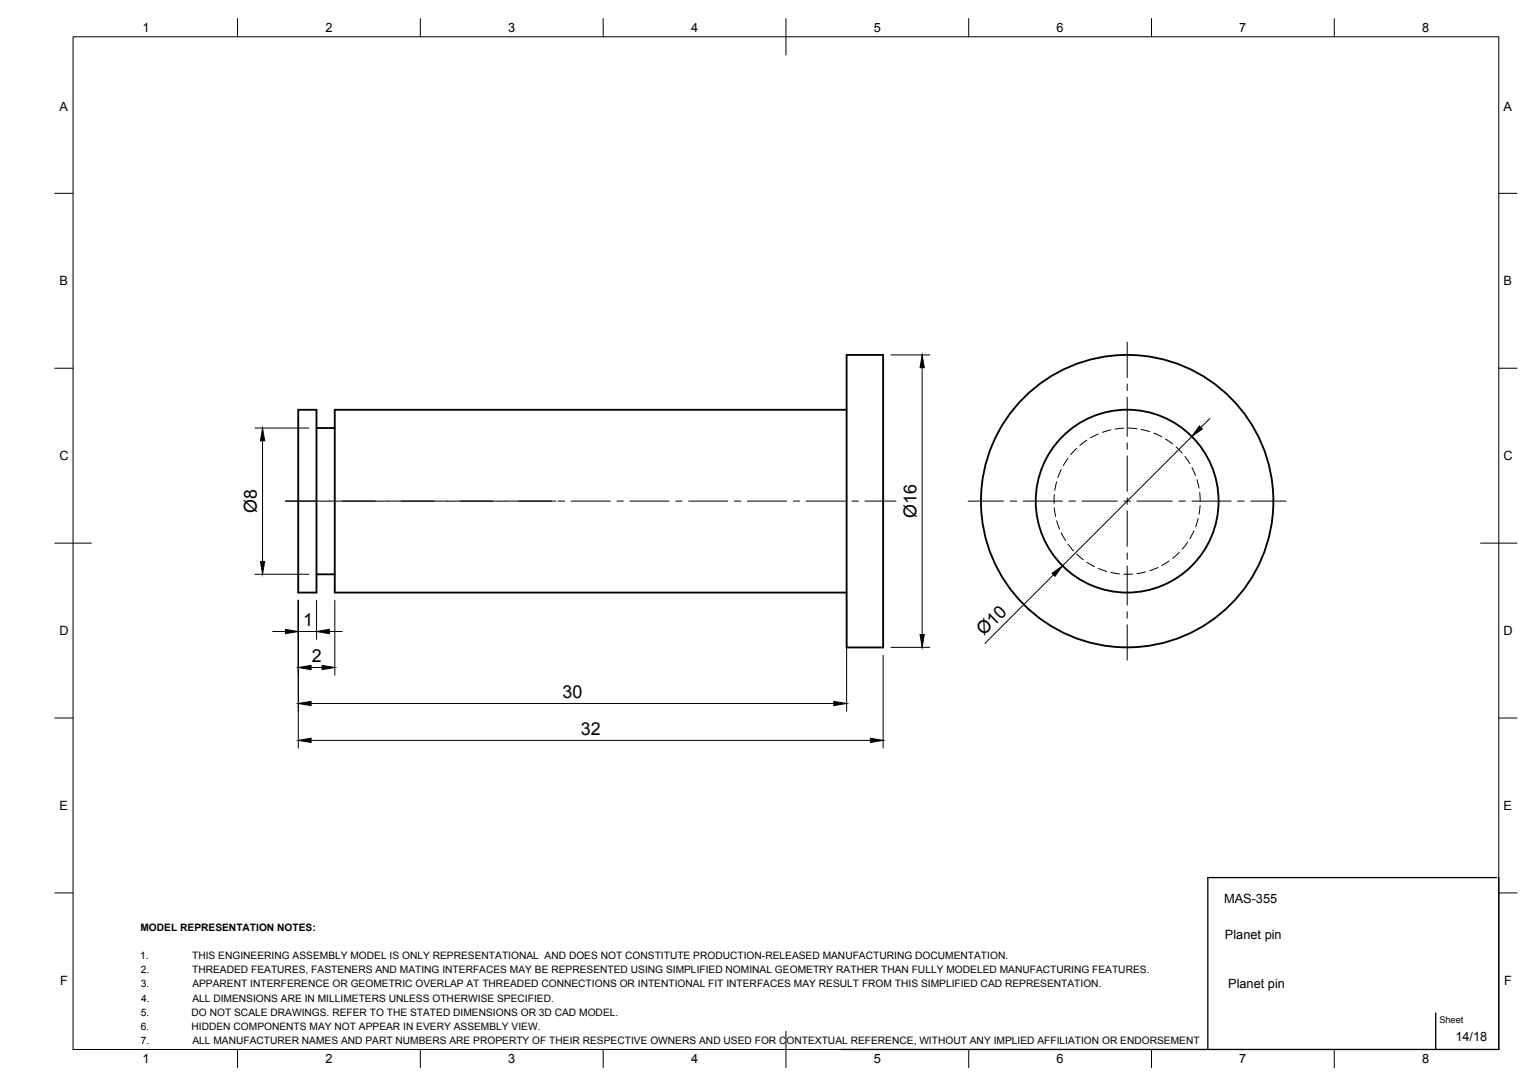
ISO-10303-21;
HEADER;
/* Generated by software containing ST-Developer
 * from STEP Tools, Inc. (www.steptools.com) 
 */

FILE_DESCRIPTION(
/* description */ ('Independent two-stage fixed-ring planetary gearbox,24/24/72 teeth,mod
ule2,20deg involutes,three planets per stage,4:1 x4:1=16:1. Native cut
-space/fillet/pattern tooth profiles derived from reusable gear blanks
; shared sun/planet/ring/carrier parts across both stages. Captured br
onze-journal input/carriers, headed retained planet pins, keyed inters
tage drive and modular keyed output interface. Native ideal gear links
; no torque, precision grade, production backlash/fits, lubrication, s
peed or life rating.'),
/* implementation_level */ '2;1');

FILE_NAME(
/* name */ 'Planet pin.step',
/* time_stamp */ '2026-11-08T19:10:00-08:00',
/* author */ (''),
/* organization */ (''),
/* preprocessor_version */ 'ST-DEVELOPER v20.2',
/* originating_system */ 'Autodesk Translation Framework v15.17.0.0',
/* authorisation */ '');

FILE_SCHEMA (('AUTOMOTIVE_DESIGN { 1 0 10303 214 3 1 1 }'));
ENDSEC;

DATA;
#10=MECHANICAL_DESIGN_GEOMETRIC_PRESENTATION_REPRESENTATION('',(#1174),#259224);
#1134=SHAPE_REPRESENTATION_RELATIONSHIP('SRR','None',#259381,#1154);
#1154=ADVANCED_BREP_SHAPE_REPRESENTATION('',(#1194),#259215);
#1174=STYLED_ITEM('',(#259488),#1194);
#1194=MANIFOLD_SOLID_BREP('Body1',#25161);
#1307=FACE_BOUND('',#4399,.T.);
#1308=FACE_BOUND('',#4401,.T.);
#1309=FACE_BOUND('',#4404,.T.);
#1663=PLANE('',#27096);
#1664=PLANE('',#27098);
#1665=PLANE('',#27102);
#1666=PLANE('',#27107);
#1667=PLANE('',#27109);
#2947=FACE_OUTER_BOUND('',#4397,.T.);
#2948=FACE_OUTER_BOUND('',#4398,.T.);
#2949=FACE_OUTER_BOUND('',#4400,.T.);
#2950=FACE_OUTER_BOUND('',#4402,.T.);
#2951=FACE_OUTER_BOUND('',#4403,.T.);
#2952=FACE_OUTER_BOUND('',#4405,.T.);
#2953=FACE_OUTER_BOUND('',#4406,.T.);
#2954=FACE_OUTER_BOUND('',#4407,.T.);
#2955=FACE_OUTER_BOUND('',#4408,.T.);
#4397=EDGE_LOOP('',(#22634,#22635,#22636,#22637));
#4398=EDGE_LOOP('',(#22638));
#4399=EDGE_LOOP('',(#22639));
#4400=EDGE_LOOP('',(#22640));
#4401=EDGE_LOOP('',(#22641));
#4402=EDGE_LOOP('',(#22642,#22643,#22644,#22645));
#4403=EDGE_LOOP('',(#22646));
#4404=EDGE_LOOP('',(#22647));
#4405=EDGE_LOOP('',(#22648,#22649,#22650,#22651));
#4406=EDGE_LOOP('',(#22652));
#4407=EDGE_LOOP('',(#22653,#22654,#22655,#22656));
#4408=EDGE_LOOP('',(#22657));
#5345=CIRCLE('',#27094,4.);
#5346=CIRCLE('',#27095,4.);
#5347=CIRCLE('',#27097,5.);
#5348=CIRCLE('',#27099,5.);
#5349=CIRCLE('',#27101,5.);
#5350=CIRCLE('',#27103,8.);
#5351=CIRCLE('',#27104,5.);
#5352=CIRCLE('',#27106,8.);
#7758=LINE('',#255948,#8943);
#7759=LINE('',#255959,#8944);
#7760=LINE('',#255967,#8945);
#7761=LINE('',#255971,#8946);
#8943=VECTOR('',#31833,4.);
#8944=VECTOR('',#31848,5.);
#8945=VECTOR('',#31857,8.);
#8946=VECTOR('',#31864,5.);
#11449=VERTEX_POINT('',#255945);
#11450=VERTEX_POINT('',#255947);
#11451=VERTEX_POINT('',#255951);
#11452=VERTEX_POINT('',#255954);
#11453=VERTEX_POINT('',#255957);
#11454=VERTEX_POINT('',#255961);
#11455=VERTEX_POINT('',#255963);
#11456=VERTEX_POINT('',#255966);
#15202=EDGE_CURVE('',#11449,#11449,#5345,.T.);
#15203=EDGE_CURVE('',#11449,#11450,#7758,.T.);
#15204=EDGE_CURVE('',#11450,#11450,#5346,.T.);
#15205=EDGE_CURVE('',#11451,#11451,#5347,.T.);
#15206=EDGE_CURVE('',#11452,#11452,#5348,.T.);
#15207=EDGE_CURVE('',#11453,#11453,#5349,.T.);
#15208=EDGE_CURVE('',#11453,#11452,#7759,.T.);
#15209=EDGE_CURVE('',#11454,#11454,#5350,.T.);
#15210=EDGE_CURVE('',#11455,#11455,#5351,.T.);
#15211=EDGE_CURVE('',#11454,#11456,#7760,.T.);
#15212=EDGE_CURVE('',#11456,#11456,#5352,.T.);
#15213=EDGE_CURVE('',#11451,#11455,#7761,.T.);
#22634=ORIENTED_EDGE('',*,*,#15202,.T.);
#22635=ORIENTED_EDGE('',*,*,#15203,.T.);
#22636=ORIENTED_EDGE('',*,*,#15204,.F.);
#22637=ORIENTED_EDGE('',*,*,#15203,.F.);
#22638=ORIENTED_EDGE('',*,*,#15205,.F.);
#22639=ORIENTED_EDGE('',*,*,#15202,.F.);
#22640=ORIENTED_EDGE('',*,*,#15206,.F.);
#22641=ORIENTED_EDGE('',*,*,#15204,.T.);
#22642=ORIENTED_EDGE('',*,*,#15207,.F.);
#22643=ORIENTED_EDGE('',*,*,#15208,.T.);
#22644=ORIENTED_EDGE('',*,*,#15206,.T.);
#22645=ORIENTED_EDGE('',*,*,#15208,.F.);
#22646=ORIENTED_EDGE('',*,*,#15209,.T.);
#22647=ORIENTED_EDGE('',*,*,#15210,.F.);
#22648=ORIENTED_EDGE('',*,*,#15209,.F.);
#22649=ORIENTED_EDGE('',*,*,#15211,.T.);
#22650=ORIENTED_EDGE('',*,*,#15212,.T.);
#22651=ORIENTED_EDGE('',*,*,#15211,.F.);
#22652=ORIENTED_EDGE('',*,*,#15212,.F.);
#22653=ORIENTED_EDGE('',*,*,#15205,.T.);
#22654=ORIENTED_EDGE('',*,*,#15213,.T.);
#22655=ORIENTED_EDGE('',*,*,#15210,.T.);
#22656=ORIENTED_EDGE('',*,*,#15213,.F.);
#22657=ORIENTED_EDGE('',*,*,#15207,.T.);
#23744=CYLINDRICAL_SURFACE('',#27093,4.);
#23745=CYLINDRICAL_SURFACE('',#27100,5.);
#23746=CYLINDRICAL_SURFACE('',#27105,8.);
#23747=CYLINDRICAL_SURFACE('',#27108,5.);
#25053=ADVANCED_FACE('',(#2947),#23744,.T.);
#25054=ADVANCED_FACE('',(#2948,#1307),#1663,.F.);
#25055=ADVANCED_FACE('',(#2949,#1308),#1664,.F.);
#25056=ADVANCED_FACE('',(#2950),#23745,.T.);
#25057=ADVANCED_FACE('',(#2951,#1309),#1665,.T.);
#25058=ADVANCED_FACE('',(#2952),#23746,.T.);
#25059=ADVANCED_FACE('',(#2953),#1666,.F.);
#25060=ADVANCED_FACE('',(#2954),#23747,.T.);
#25061=ADVANCED_FACE('',(#2955),#1667,.T.);
#25161=CLOSED_SHELL('',(#25053,#25054,#25055,#25056,#25057,#25058,#25059,
#25060,#25061));
#27092=AXIS2_PLACEMENT_3D('',#255943,#31827,#31828);
#27093=AXIS2_PLACEMENT_3D('',#255944,#31829,#31830);
#27094=AXIS2_PLACEMENT_3D('',#255946,#31831,#31832);
#27095=AXIS2_PLACEMENT_3D('',#255949,#31834,#31835);
#27096=AXIS2_PLACEMENT_3D('',#255950,#31836,#31837);
#27097=AXIS2_PLACEMENT_3D('',#255952,#31838,#31839);
#27098=AXIS2_PLACEMENT_3D('',#255953,#31840,#31841);
#27099=AXIS2_PLACEMENT_3D('',#255955,#31842,#31843);
#27100=AXIS2_PLACEMENT_3D('',#255956,#31844,#31845);
#27101=AXIS2_PLACEMENT_3D('',#255958,#31846,#31847);
#27102=AXIS2_PLACEMENT_3D('',#255960,#31849,#31850);
#27103=AXIS2_PLACEMENT_3D('',#255962,#31851,#31852);
#27104=AXIS2_PLACEMENT_3D('',#255964,#31853,#31854);
#27105=AXIS2_PLACEMENT_3D('',#255965,#31855,#31856);
#27106=AXIS2_PLACEMENT_3D('',#255968,#31858,#31859);
#27107=AXIS2_PLACEMENT_3D('',#255969,#31860,#31861);
#27108=AXIS2_PLACEMENT_3D('',#255970,#31862,#31863);
#27109=AXIS2_PLACEMENT_3D('',#255972,#31865,#31866);
#31827=DIRECTION('axis',(0.,0.,1.));
#31828=DIRECTION('refdir',(1.,0.,0.));
#31829=DIRECTION('center_axis',(0.,0.,1.));
#31830=DIRECTION('ref_axis',(1.,0.,0.));
#31831=DIRECTION('center_axis',(0.,0.,1.));
#31832=DIRECTION('ref_axis',(1.,0.,0.));
#31833=DIRECTION('',(0.,0.,1.));
#31834=DIRECTION('center_axis',(0.,0.,1.));
#31835=DIRECTION('ref_axis',(1.,0.,0.));
#31836=DIRECTION('center_axis',(0.,0.,-1.));
#31837=DIRECTION('ref_axis',(-1.,0.,0.));
#31838=DIRECTION('center_axis',(0.,0.,-1.));
#31839=DIRECTION('ref_axis',(1.,0.,0.));
#31840=DIRECTION('center_axis',(0.,0.,1.));
#31841=DIRECTION('ref_axis',(1.,0.,0.));
#31842=DIRECTION('center_axis',(0.,0.,1.));
#31843=DIRECTION('ref_axis',(1.,0.,0.));
#31844=DIRECTION('center_axis',(0.,0.,1.));
#31845=DIRECTION('ref_axis',(1.,0.,0.));
#31846=DIRECTION('center_axis',(0.,0.,1.));
#31847=DIRECTION('ref_axis',(1.,0.,0.));
#31848=DIRECTION('',(0.,0.,-1.));
#31849=DIRECTION('center_axis',(0.,0.,1.));
#31850=DIRECTION('ref_axis',(1.,0.,0.));
#31851=DIRECTION('center_axis',(0.,0.,1.));
#31852=DIRECTION('ref_axis',(1.,0.,0.));
#31853=DIRECTION('center_axis',(0.,0.,1.));
#31854=DIRECTION('ref_axis',(1.,0.,0.));
#31855=DIRECTION('center_axis',(0.,0.,1.));
#31856=DIRECTION('ref_axis',(1.,0.,0.));
#31857=DIRECTION('',(0.,0.,-1.));
#31858=DIRECTION('center_axis',(0.,0.,1.));
#31859=DIRECTION('ref_axis',(1.,0.,0.));
#31860=DIRECTION('center_axis',(0.,0.,1.));
#31861=DIRECTION('ref_axis',(1.,0.,0.));
#31862=DIRECTION('center_axis',(0.,0.,1.));
#31863=DIRECTION('ref_axis',(1.,0.,0.));
#31864=DIRECTION('',(0.,0.,-1.));
#31865=DIRECTION('center_axis',(0.,0.,1.));
#31866=DIRECTION('ref_axis',(1.,0.,0.));
#255943=CARTESIAN_POINT('',(0.,0.,0.));
#255944=CARTESIAN_POINT('Origin',(0.,0.,28.5));
#255945=CARTESIAN_POINT('',(-4.,-4.89858719658941E-16,28.));
#255946=CARTESIAN_POINT('Origin',(0.,0.,28.));
#255947=CARTESIAN_POINT('',(-4.,-4.89858719658941E-16,29.));
#255948=CARTESIAN_POINT('',(-4.,-4.89858719658941E-16,28.5));
#255949=CARTESIAN_POINT('Origin',(0.,0.,29.));
#255950=CARTESIAN_POINT('Origin',(8.,0.,28.));
#255951=CARTESIAN_POINT('',(-5.,6.12323399573677E-16,28.));
#255952=CARTESIAN_POINT('Origin',(0.,0.,28.));
#255953=CARTESIAN_POINT('Origin',(4.,0.,29.));
#255954=CARTESIAN_POINT('',(-5.,-6.12323399573677E-16,29.));
#255955=CARTESIAN_POINT('Origin',(0.,0.,29.));
#255956=CARTESIAN_POINT('Origin',(0.,0.,0.));
#255957=CARTESIAN_POINT('',(-5.,-6.12323399573677E-16,30.));
#255958=CARTESIAN_POINT('Origin',(0.,0.,30.));
#255959=CARTESIAN_POINT('',(-5.,-6.12323399573677E-16,0.));
#255960=CARTESIAN_POINT('Origin',(0.,0.,0.));
#255961=CARTESIAN_POINT('',(-8.,-9.79717439317883E-16,0.));
#255962=CARTESIAN_POINT('Origin',(0.,0.,0.));
#255963=CARTESIAN_POINT('',(-5.,-6.12323399573677E-16,0.));
#255964=CARTESIAN_POINT('Origin',(0.,0.,0.));
#255965=CARTESIAN_POINT('Origin',(0.,0.,-2.));
#255966=CARTESIAN_POINT('',(-8.,-9.79717439317883E-16,-2.));
#255967=CARTESIAN_POINT('',(-8.,-9.79717439317883E-16,-2.));
#255968=CARTESIAN_POINT('Origin',(0.,0.,-2.));
#255969=CARTESIAN_POINT('Origin',(0.,0.,-2.));
#255970=CARTESIAN_POINT('Origin',(0.,0.,0.));
#255971=CARTESIAN_POINT('',(-5.,-6.12323399573677E-16,0.));
#255972=CARTESIAN_POINT('Origin',(0.,0.,30.));
#259193=UNCERTAINTY_MEASURE_WITH_UNIT(LENGTH_MEASURE(0.01),#259225,
'DISTANCE_ACCURACY_VALUE',
'Maximum model space distance between geometric entities at asserted c
onnectivities');
#259202=UNCERTAINTY_MEASURE_WITH_UNIT(LENGTH_MEASURE(0.01),#259225,
'DISTANCE_ACCURACY_VALUE',
'Maximum model space distance between geometric entities at asserted c
onnectivities');
#259215=(
GEOMETRIC_REPRESENTATION_CONTEXT(3)
GLOBAL_UNCERTAINTY_ASSIGNED_CONTEXT((#259193))
GLOBAL_UNIT_ASSIGNED_CONTEXT((#259225,#259227,#259228))
REPRESENTATION_CONTEXT('','3D')
);
#259224=(
GEOMETRIC_REPRESENTATION_CONTEXT(3)
GLOBAL_UNCERTAINTY_ASSIGNED_CONTEXT((#259202))
GLOBAL_UNIT_ASSIGNED_CONTEXT((#259225,#259227,#259228))
REPRESENTATION_CONTEXT('','3D')
);
#259225=(
LENGTH_UNIT()
NAMED_UNIT(*)
SI_UNIT(.MILLI.,.METRE.)
);
#259227=(
NAMED_UNIT(*)
PLANE_ANGLE_UNIT()
SI_UNIT($,.RADIAN.)
);
#259228=(
NAMED_UNIT(*)
SI_UNIT($,.STERADIAN.)
SOLID_ANGLE_UNIT()
);
#259241=SHAPE_DEFINITION_REPRESENTATION(#259262,#259381);
#259262=PRODUCT_DEFINITION_SHAPE('',$,#259403);
#259381=SHAPE_REPRESENTATION('',(#27092),#259215);
#259390=PRODUCT_DEFINITION_CONTEXT('part definition',#259455,'design');
#259403=PRODUCT_DEFINITION('Planet pin','Planet pin',#259424,#259390);
#259424=PRODUCT_DEFINITION_FORMATION('',$,#259469);
#259455=APPLICATION_CONTEXT(
'Core Data for Automotive Mechanical Design Process');
#259456=PRODUCT_CONTEXT('part definition',#259455,'mechanical');
#259469=PRODUCT('Planet pin','Planet pin',$,(#259456));
#259488=PRESENTATION_STYLE_ASSIGNMENT((#259503));
#259503=SURFACE_STYLE_USAGE(.BOTH.,#259518);
#259518=SURFACE_SIDE_STYLE('',(#259533));
#259533=SURFACE_STYLE_FILL_AREA(#259548);
#259548=FILL_AREA_STYLE('Pin gray',(#259563));
#259563=FILL_AREA_STYLE_COLOUR('Pin gray',#259578);
#259578=COLOUR_RGB('Pin gray',0.576470588235294,0.615686274509804,0.666666666666667);
ENDSEC;
END-ISO-10303-21;
